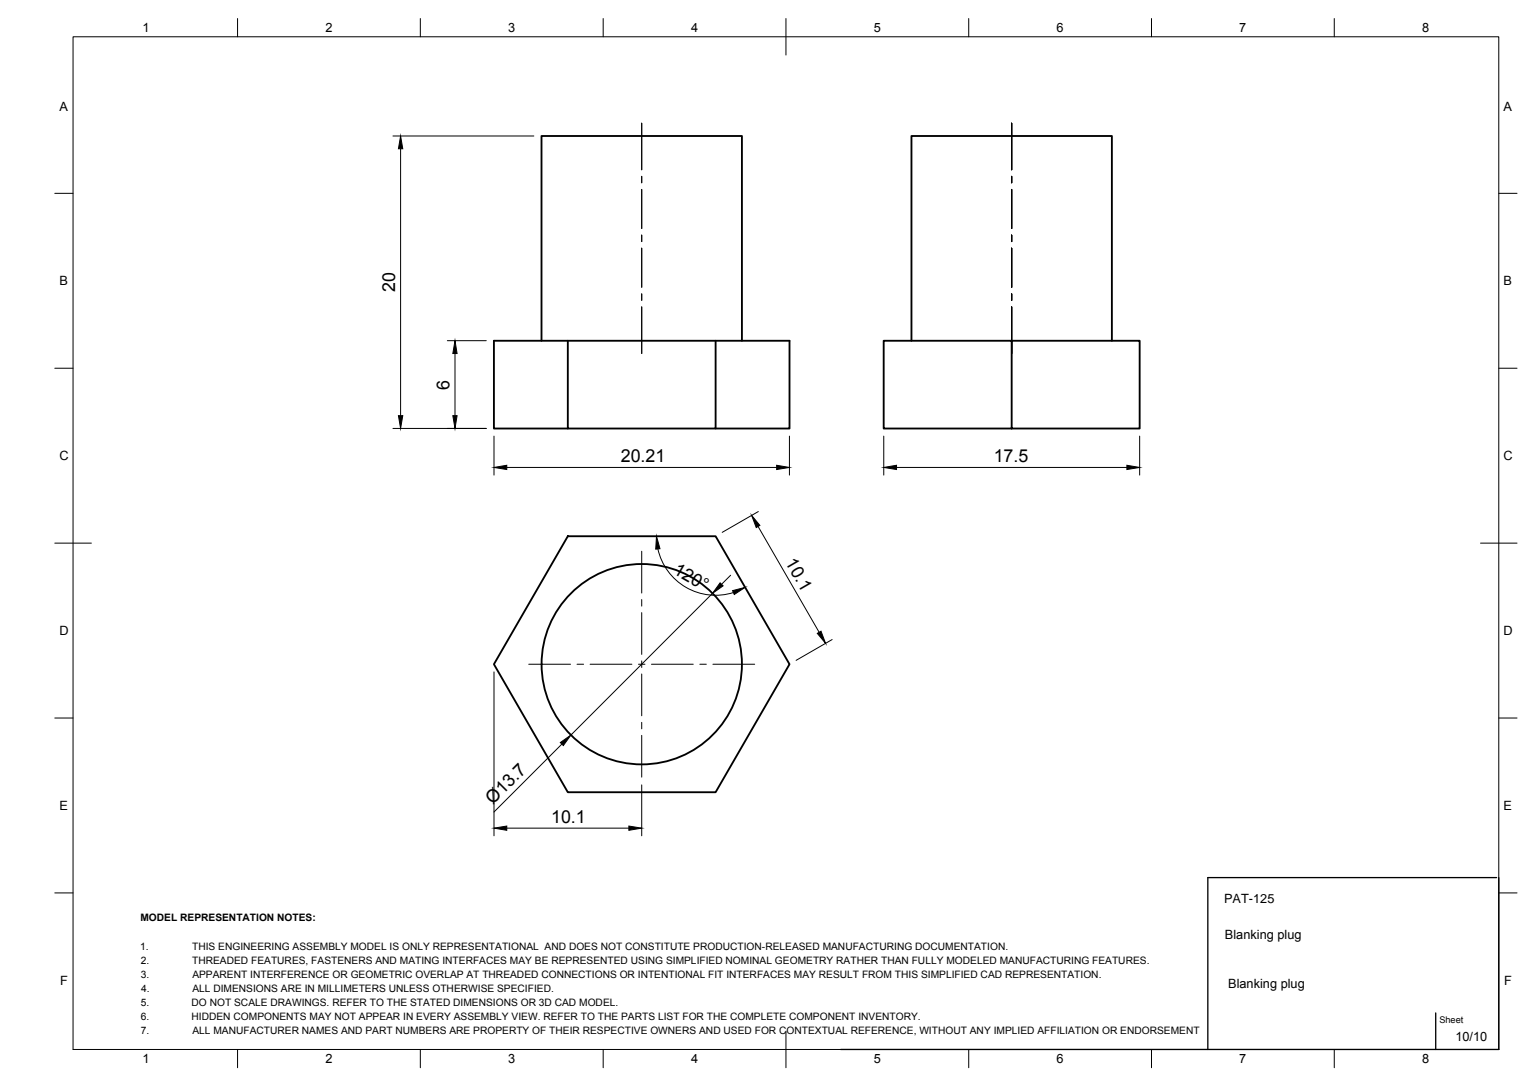
ISO-10303-21;
HEADER;
/* Generated by software containing ST-Developer
 * from STEP Tools, Inc. (www.steptools.com) 
 */

FILE_DESCRIPTION(
/* description */ ('Y-strainer with drain'),
/* implementation_level */ '2;1');

FILE_NAME(
/* name */ 'Blanking plug.step',
/* time_stamp */ '2026-10-28T00:41:55-07:00',
/* author */ (''),
/* organization */ (''),
/* preprocessor_version */ 'ST-DEVELOPER v20.2',
/* originating_system */ 'Autodesk Translation Framework v15.17.0.0',
/* authorisation */ '');

FILE_SCHEMA (('AUTOMOTIVE_DESIGN { 1 0 10303 214 3 1 1 }'));
ENDSEC;

DATA;
#10=MECHANICAL_DESIGN_GEOMETRIC_PRESENTATION_REPRESENTATION('',(#101),#8864);
#83=SHAPE_REPRESENTATION_RELATIONSHIP('SRR','None',#8915,#92);
#92=ADVANCED_BREP_SHAPE_REPRESENTATION('',(#109),#8863);
#101=STYLED_ITEM('',(#9047),#109);
#109=MANIFOLD_SOLID_BREP('Body1',#3392);
#455=FACE_BOUND('',#951,.T.);
#511=PLANE('',#3745);
#512=PLANE('',#3747);
#513=PLANE('',#3748);
#514=PLANE('',#3749);
#515=PLANE('',#3750);
#516=PLANE('',#3751);
#517=PLANE('',#3752);
#518=PLANE('',#3753);
#519=PLANE('',#3756);
#662=FACE_OUTER_BOUND('',#950,.T.);
#663=FACE_OUTER_BOUND('',#952,.T.);
#664=FACE_OUTER_BOUND('',#953,.T.);
#665=FACE_OUTER_BOUND('',#954,.T.);
#666=FACE_OUTER_BOUND('',#955,.T.);
#667=FACE_OUTER_BOUND('',#956,.T.);
#668=FACE_OUTER_BOUND('',#957,.T.);
#669=FACE_OUTER_BOUND('',#958,.T.);
#670=FACE_OUTER_BOUND('',#959,.T.);
#671=FACE_OUTER_BOUND('',#960,.T.);
#950=EDGE_LOOP('',(#3098,#3099,#3100,#3101,#3102,#3103));
#951=EDGE_LOOP('',(#3104));
#952=EDGE_LOOP('',(#3105,#3106,#3107,#3108));
#953=EDGE_LOOP('',(#3109,#3110,#3111,#3112));
#954=EDGE_LOOP('',(#3113,#3114,#3115,#3116));
#955=EDGE_LOOP('',(#3117,#3118,#3119,#3120));
#956=EDGE_LOOP('',(#3121,#3122,#3123,#3124));
#957=EDGE_LOOP('',(#3125,#3126,#3127,#3128));
#958=EDGE_LOOP('',(#3129,#3130,#3131,#3132,#3133,#3134));
#959=EDGE_LOOP('',(#3135,#3136,#3137,#3138));
#960=EDGE_LOOP('',(#3139));
#1105=LINE('',#8785,#1268);
#1106=LINE('',#8787,#1269);
#1107=LINE('',#8789,#1270);
#1108=LINE('',#8791,#1271);
#1109=LINE('',#8793,#1272);
#1110=LINE('',#8794,#1273);
#1111=LINE('',#8799,#1274);
#1112=LINE('',#8801,#1275);
#1113=LINE('',#8802,#1276);
#1114=LINE('',#8805,#1277);
#1115=LINE('',#8806,#1278);
#1116=LINE('',#8809,#1279);
#1117=LINE('',#8810,#1280);
#1118=LINE('',#8813,#1281);
#1119=LINE('',#8814,#1282);
#1120=LINE('',#8817,#1283);
#1121=LINE('',#8818,#1284);
#1122=LINE('',#8820,#1285);
#1123=LINE('',#8824,#1286);
#1268=VECTOR('',#4421,1.);
#1269=VECTOR('',#4422,1.);
#1270=VECTOR('',#4423,1.);
#1271=VECTOR('',#4424,1.);
#1272=VECTOR('',#4425,1.);
#1273=VECTOR('',#4426,1.);
#1274=VECTOR('',#4431,1.);
#1275=VECTOR('',#4432,1.);
#1276=VECTOR('',#4433,1.);
#1277=VECTOR('',#4436,1.);
#1278=VECTOR('',#4437,1.);
#1279=VECTOR('',#4440,1.);
#1280=VECTOR('',#4441,1.);
#1281=VECTOR('',#4444,1.);
#1282=VECTOR('',#4445,1.);
#1283=VECTOR('',#4448,1.);
#1284=VECTOR('',#4449,1.);
#1285=VECTOR('',#4452,1.);
#1286=VECTOR('',#4457,0.685);
#1377=CIRCLE('',#3746,0.685);
#1378=CIRCLE('',#3755,0.685);
#1707=VERTEX_POINT('',#8783);
#1708=VERTEX_POINT('',#8784);
#1709=VERTEX_POINT('',#8786);
#1710=VERTEX_POINT('',#8788);
#1711=VERTEX_POINT('',#8790);
#1712=VERTEX_POINT('',#8792);
#1713=VERTEX_POINT('',#8795);
#1714=VERTEX_POINT('',#8798);
#1715=VERTEX_POINT('',#8800);
#1716=VERTEX_POINT('',#8804);
#1717=VERTEX_POINT('',#8808);
#1718=VERTEX_POINT('',#8812);
#1719=VERTEX_POINT('',#8816);
#1720=VERTEX_POINT('',#8823);
#2173=EDGE_CURVE('',#1707,#1708,#1105,.T.);
#2174=EDGE_CURVE('',#1709,#1707,#1106,.T.);
#2175=EDGE_CURVE('',#1710,#1709,#1107,.T.);
#2176=EDGE_CURVE('',#1711,#1710,#1108,.T.);
#2177=EDGE_CURVE('',#1712,#1711,#1109,.T.);
#2178=EDGE_CURVE('',#1708,#1712,#1110,.T.);
#2179=EDGE_CURVE('',#1713,#1713,#1377,.T.);
#2180=EDGE_CURVE('',#1707,#1714,#1111,.T.);
#2181=EDGE_CURVE('',#1715,#1714,#1112,.T.);
#2182=EDGE_CURVE('',#1709,#1715,#1113,.T.);
#2183=EDGE_CURVE('',#1716,#1715,#1114,.T.);
#2184=EDGE_CURVE('',#1710,#1716,#1115,.T.);
#2185=EDGE_CURVE('',#1717,#1716,#1116,.T.);
#2186=EDGE_CURVE('',#1711,#1717,#1117,.T.);
#2187=EDGE_CURVE('',#1718,#1717,#1118,.T.);
#2188=EDGE_CURVE('',#1712,#1718,#1119,.T.);
#2189=EDGE_CURVE('',#1719,#1718,#1120,.T.);
#2190=EDGE_CURVE('',#1708,#1719,#1121,.T.);
#2191=EDGE_CURVE('',#1714,#1719,#1122,.T.);
#2192=EDGE_CURVE('',#1713,#1720,#1123,.T.);
#2193=EDGE_CURVE('',#1720,#1720,#1378,.T.);
#3098=ORIENTED_EDGE('',*,*,#2173,.F.);
#3099=ORIENTED_EDGE('',*,*,#2174,.F.);
#3100=ORIENTED_EDGE('',*,*,#2175,.F.);
#3101=ORIENTED_EDGE('',*,*,#2176,.F.);
#3102=ORIENTED_EDGE('',*,*,#2177,.F.);
#3103=ORIENTED_EDGE('',*,*,#2178,.F.);
#3104=ORIENTED_EDGE('',*,*,#2179,.T.);
#3105=ORIENTED_EDGE('',*,*,#2174,.T.);
#3106=ORIENTED_EDGE('',*,*,#2180,.T.);
#3107=ORIENTED_EDGE('',*,*,#2181,.F.);
#3108=ORIENTED_EDGE('',*,*,#2182,.F.);
#3109=ORIENTED_EDGE('',*,*,#2175,.T.);
#3110=ORIENTED_EDGE('',*,*,#2182,.T.);
#3111=ORIENTED_EDGE('',*,*,#2183,.F.);
#3112=ORIENTED_EDGE('',*,*,#2184,.F.);
#3113=ORIENTED_EDGE('',*,*,#2176,.T.);
#3114=ORIENTED_EDGE('',*,*,#2184,.T.);
#3115=ORIENTED_EDGE('',*,*,#2185,.F.);
#3116=ORIENTED_EDGE('',*,*,#2186,.F.);
#3117=ORIENTED_EDGE('',*,*,#2177,.T.);
#3118=ORIENTED_EDGE('',*,*,#2186,.T.);
#3119=ORIENTED_EDGE('',*,*,#2187,.F.);
#3120=ORIENTED_EDGE('',*,*,#2188,.F.);
#3121=ORIENTED_EDGE('',*,*,#2178,.T.);
#3122=ORIENTED_EDGE('',*,*,#2188,.T.);
#3123=ORIENTED_EDGE('',*,*,#2189,.F.);
#3124=ORIENTED_EDGE('',*,*,#2190,.F.);
#3125=ORIENTED_EDGE('',*,*,#2173,.T.);
#3126=ORIENTED_EDGE('',*,*,#2190,.T.);
#3127=ORIENTED_EDGE('',*,*,#2191,.F.);
#3128=ORIENTED_EDGE('',*,*,#2180,.F.);
#3129=ORIENTED_EDGE('',*,*,#2191,.T.);
#3130=ORIENTED_EDGE('',*,*,#2189,.T.);
#3131=ORIENTED_EDGE('',*,*,#2187,.T.);
#3132=ORIENTED_EDGE('',*,*,#2185,.T.);
#3133=ORIENTED_EDGE('',*,*,#2183,.T.);
#3134=ORIENTED_EDGE('',*,*,#2181,.T.);
#3135=ORIENTED_EDGE('',*,*,#2179,.F.);
#3136=ORIENTED_EDGE('',*,*,#2192,.T.);
#3137=ORIENTED_EDGE('',*,*,#2193,.T.);
#3138=ORIENTED_EDGE('',*,*,#2192,.F.);
#3139=ORIENTED_EDGE('',*,*,#2193,.F.);
#3230=CYLINDRICAL_SURFACE('',#3754,0.685);
#3373=ADVANCED_FACE('',(#662,#455),#511,.F.);
#3374=ADVANCED_FACE('',(#663),#512,.T.);
#3375=ADVANCED_FACE('',(#664),#513,.T.);
#3376=ADVANCED_FACE('',(#665),#514,.T.);
#3377=ADVANCED_FACE('',(#666),#515,.T.);
#3378=ADVANCED_FACE('',(#667),#516,.T.);
#3379=ADVANCED_FACE('',(#668),#517,.T.);
#3380=ADVANCED_FACE('',(#669),#518,.T.);
#3381=ADVANCED_FACE('',(#670),#3230,.T.);
#3382=ADVANCED_FACE('',(#671),#519,.F.);
#3392=CLOSED_SHELL('',(#3373,#3374,#3375,#3376,#3377,#3378,#3379,#3380,
#3381,#3382));
#3744=AXIS2_PLACEMENT_3D('',#8781,#4417,#4418);
#3745=AXIS2_PLACEMENT_3D('',#8782,#4419,#4420);
#3746=AXIS2_PLACEMENT_3D('',#8796,#4427,#4428);
#3747=AXIS2_PLACEMENT_3D('',#8797,#4429,#4430);
#3748=AXIS2_PLACEMENT_3D('',#8803,#4434,#4435);
#3749=AXIS2_PLACEMENT_3D('',#8807,#4438,#4439);
#3750=AXIS2_PLACEMENT_3D('',#8811,#4442,#4443);
#3751=AXIS2_PLACEMENT_3D('',#8815,#4446,#4447);
#3752=AXIS2_PLACEMENT_3D('',#8819,#4450,#4451);
#3753=AXIS2_PLACEMENT_3D('',#8821,#4453,#4454);
#3754=AXIS2_PLACEMENT_3D('',#8822,#4455,#4456);
#3755=AXIS2_PLACEMENT_3D('',#8825,#4458,#4459);
#3756=AXIS2_PLACEMENT_3D('',#8826,#4460,#4461);
#4417=DIRECTION('axis',(0.,0.,1.));
#4418=DIRECTION('refdir',(1.,0.,0.));
#4419=DIRECTION('center_axis',(1.,0.,0.));
#4420=DIRECTION('ref_axis',(0.,0.,-1.));
#4421=DIRECTION('',(0.,0.5,0.866025403784439));
#4422=DIRECTION('',(0.,1.,-4.39534328316243E-16));
#4423=DIRECTION('',(0.,0.5,-0.866025403784439));
#4424=DIRECTION('',(0.,-0.5,-0.866025403784439));
#4425=DIRECTION('',(0.,-1.,0.));
#4426=DIRECTION('',(0.,-0.5,0.866025403784439));
#4427=DIRECTION('center_axis',(1.,0.,0.));
#4428=DIRECTION('ref_axis',(0.,0.,-1.));
#4429=DIRECTION('center_axis',(0.,-4.39534328316243E-16,-1.));
#4430=DIRECTION('ref_axis',(0.,1.,-4.39534328316243E-16));
#4431=DIRECTION('',(1.,0.,0.));
#4432=DIRECTION('',(0.,1.,-4.39534328316243E-16));
#4433=DIRECTION('',(1.,0.,0.));
#4434=DIRECTION('center_axis',(0.,-0.866025403784439,-0.5));
#4435=DIRECTION('ref_axis',(0.,0.5,-0.866025403784439));
#4436=DIRECTION('',(0.,0.5,-0.866025403784439));
#4437=DIRECTION('',(1.,0.,0.));
#4438=DIRECTION('center_axis',(0.,-0.866025403784439,0.5));
#4439=DIRECTION('ref_axis',(0.,-0.5,-0.866025403784439));
#4440=DIRECTION('',(0.,-0.5,-0.866025403784439));
#4441=DIRECTION('',(1.,0.,0.));
#4442=DIRECTION('center_axis',(0.,0.,1.));
#4443=DIRECTION('ref_axis',(0.,-1.,0.));
#4444=DIRECTION('',(0.,-1.,0.));
#4445=DIRECTION('',(1.,0.,0.));
#4446=DIRECTION('center_axis',(0.,0.866025403784439,0.5));
#4447=DIRECTION('ref_axis',(0.,-0.5,0.866025403784439));
#4448=DIRECTION('',(0.,-0.5,0.866025403784439));
#4449=DIRECTION('',(1.,0.,0.));
#4450=DIRECTION('center_axis',(0.,0.866025403784439,-0.5));
#4451=DIRECTION('ref_axis',(0.,0.5,0.866025403784439));
#4452=DIRECTION('',(0.,0.5,0.866025403784439));
#4453=DIRECTION('center_axis',(1.,0.,0.));
#4454=DIRECTION('ref_axis',(0.,0.,-1.));
#4455=DIRECTION('center_axis',(1.,0.,0.));
#4456=DIRECTION('ref_axis',(0.,0.,-1.));
#4457=DIRECTION('',(-1.,0.,0.));
#4458=DIRECTION('center_axis',(1.,0.,0.));
#4459=DIRECTION('ref_axis',(0.,0.,-1.));
#4460=DIRECTION('center_axis',(1.,0.,0.));
#4461=DIRECTION('ref_axis',(0.,0.,-1.));
#8781=CARTESIAN_POINT('',(0.,0.,0.));
#8782=CARTESIAN_POINT('Origin',(5.5,0.,3.5));
#8783=CARTESIAN_POINT('',(5.5,0.505181485540923,2.625));
#8784=CARTESIAN_POINT('',(5.5,1.01036297108185,3.5));
#8785=CARTESIAN_POINT('',(5.5,0.505181485540923,2.625));
#8786=CARTESIAN_POINT('',(5.5,-0.505181485540923,2.625));
#8787=CARTESIAN_POINT('',(5.5,-0.505181485540923,2.625));
#8788=CARTESIAN_POINT('',(5.5,-1.01036297108185,3.5));
#8789=CARTESIAN_POINT('',(5.5,-1.01036297108185,3.5));
#8790=CARTESIAN_POINT('',(5.5,-0.505181485540922,4.375));
#8791=CARTESIAN_POINT('',(5.5,-0.505181485540922,4.375));
#8792=CARTESIAN_POINT('',(5.5,0.505181485540923,4.375));
#8793=CARTESIAN_POINT('',(5.5,0.505181485540923,4.375));
#8794=CARTESIAN_POINT('',(5.5,1.01036297108185,3.5));
#8795=CARTESIAN_POINT('',(5.5,-8.38883057415937E-17,4.185));
#8796=CARTESIAN_POINT('Origin',(5.5,0.,3.5));
#8797=CARTESIAN_POINT('Origin',(5.5,-0.505181485540923,2.625));
#8798=CARTESIAN_POINT('',(6.1,0.505181485540923,2.625));
#8799=CARTESIAN_POINT('',(5.5,0.505181485540923,2.625));
#8800=CARTESIAN_POINT('',(6.1,-0.505181485540923,2.625));
#8801=CARTESIAN_POINT('',(6.1,-0.505181485540923,2.625));
#8802=CARTESIAN_POINT('',(5.5,-0.505181485540923,2.625));
#8803=CARTESIAN_POINT('Origin',(5.5,-1.01036297108185,3.5));
#8804=CARTESIAN_POINT('',(6.1,-1.01036297108185,3.5));
#8805=CARTESIAN_POINT('',(6.1,-1.01036297108185,3.5));
#8806=CARTESIAN_POINT('',(5.5,-1.01036297108185,3.5));
#8807=CARTESIAN_POINT('Origin',(5.5,-0.505181485540922,4.375));
#8808=CARTESIAN_POINT('',(6.1,-0.505181485540922,4.375));
#8809=CARTESIAN_POINT('',(6.1,-0.505181485540922,4.375));
#8810=CARTESIAN_POINT('',(5.5,-0.505181485540922,4.375));
#8811=CARTESIAN_POINT('Origin',(5.5,0.505181485540923,4.375));
#8812=CARTESIAN_POINT('',(6.1,0.505181485540923,4.375));
#8813=CARTESIAN_POINT('',(6.1,0.505181485540923,4.375));
#8814=CARTESIAN_POINT('',(5.5,0.505181485540923,4.375));
#8815=CARTESIAN_POINT('Origin',(5.5,1.01036297108185,3.5));
#8816=CARTESIAN_POINT('',(6.1,1.01036297108185,3.5));
#8817=CARTESIAN_POINT('',(6.1,1.01036297108185,3.5));
#8818=CARTESIAN_POINT('',(5.5,1.01036297108185,3.5));
#8819=CARTESIAN_POINT('Origin',(5.5,0.505181485540923,2.625));
#8820=CARTESIAN_POINT('',(6.1,0.505181485540923,2.625));
#8821=CARTESIAN_POINT('Origin',(6.1,0.,3.5));
#8822=CARTESIAN_POINT('Origin',(4.1,0.,3.5));
#8823=CARTESIAN_POINT('',(4.1,-8.38883057415937E-17,4.185));
#8824=CARTESIAN_POINT('',(4.1,-8.38883057415937E-17,4.185));
#8825=CARTESIAN_POINT('Origin',(4.1,0.,3.5));
#8826=CARTESIAN_POINT('Origin',(4.1,0.,3.5));
#8851=UNCERTAINTY_MEASURE_WITH_UNIT(LENGTH_MEASURE(0.001),#8865,
'DISTANCE_ACCURACY_VALUE',
'Maximum model space distance between geometric entities at asserted c
onnectivities');
#8852=UNCERTAINTY_MEASURE_WITH_UNIT(LENGTH_MEASURE(0.001),#8865,
'DISTANCE_ACCURACY_VALUE',
'Maximum model space distance between geometric entities at asserted c
onnectivities');
#8863=(
GEOMETRIC_REPRESENTATION_CONTEXT(3)
GLOBAL_UNCERTAINTY_ASSIGNED_CONTEXT((#8851))
GLOBAL_UNIT_ASSIGNED_CONTEXT((#8865,#8867,#8868))
REPRESENTATION_CONTEXT('','3D')
);
#8864=(
GEOMETRIC_REPRESENTATION_CONTEXT(3)
GLOBAL_UNCERTAINTY_ASSIGNED_CONTEXT((#8852))
GLOBAL_UNIT_ASSIGNED_CONTEXT((#8865,#8867,#8868))
REPRESENTATION_CONTEXT('','3D')
);
#8865=(
LENGTH_UNIT()
NAMED_UNIT(*)
SI_UNIT(.CENTI.,.METRE.)
);
#8867=(
NAMED_UNIT(*)
PLANE_ANGLE_UNIT()
SI_UNIT($,.RADIAN.)
);
#8868=(
NAMED_UNIT(*)
SI_UNIT($,.STERADIAN.)
SOLID_ANGLE_UNIT()
);
#8879=SHAPE_DEFINITION_REPRESENTATION(#8890,#8915);
#8890=PRODUCT_DEFINITION_SHAPE('',$,#8927);
#8915=SHAPE_REPRESENTATION('',(#3744),#8863);
#8916=PRODUCT_DEFINITION_CONTEXT('part definition',#8951,'design');
#8927=PRODUCT_DEFINITION('Blanking plug','Blanking plug',#8938,#8916);
#8938=PRODUCT_DEFINITION_FORMATION('',$,#8963);
#8951=APPLICATION_CONTEXT(
'Core Data for Automotive Mechanical Design Process');
#8952=PRODUCT_CONTEXT('part definition',#8951,'mechanical');
#8963=PRODUCT('Blanking plug','Blanking plug','Blanking plug',(#8952));
#9041=COLOUR_RGB('Off White',0.89,0.88,0.83);
#9042=FILL_AREA_STYLE_COLOUR('',#9041);
#9043=FILL_AREA_STYLE('',(#9042));
#9044=SURFACE_STYLE_FILL_AREA(#9043);
#9045=SURFACE_SIDE_STYLE('',(#9044));
#9046=SURFACE_STYLE_USAGE(.BOTH.,#9045);
#9047=PRESENTATION_STYLE_ASSIGNMENT((#9046));
ENDSEC;
END-ISO-10303-21;
